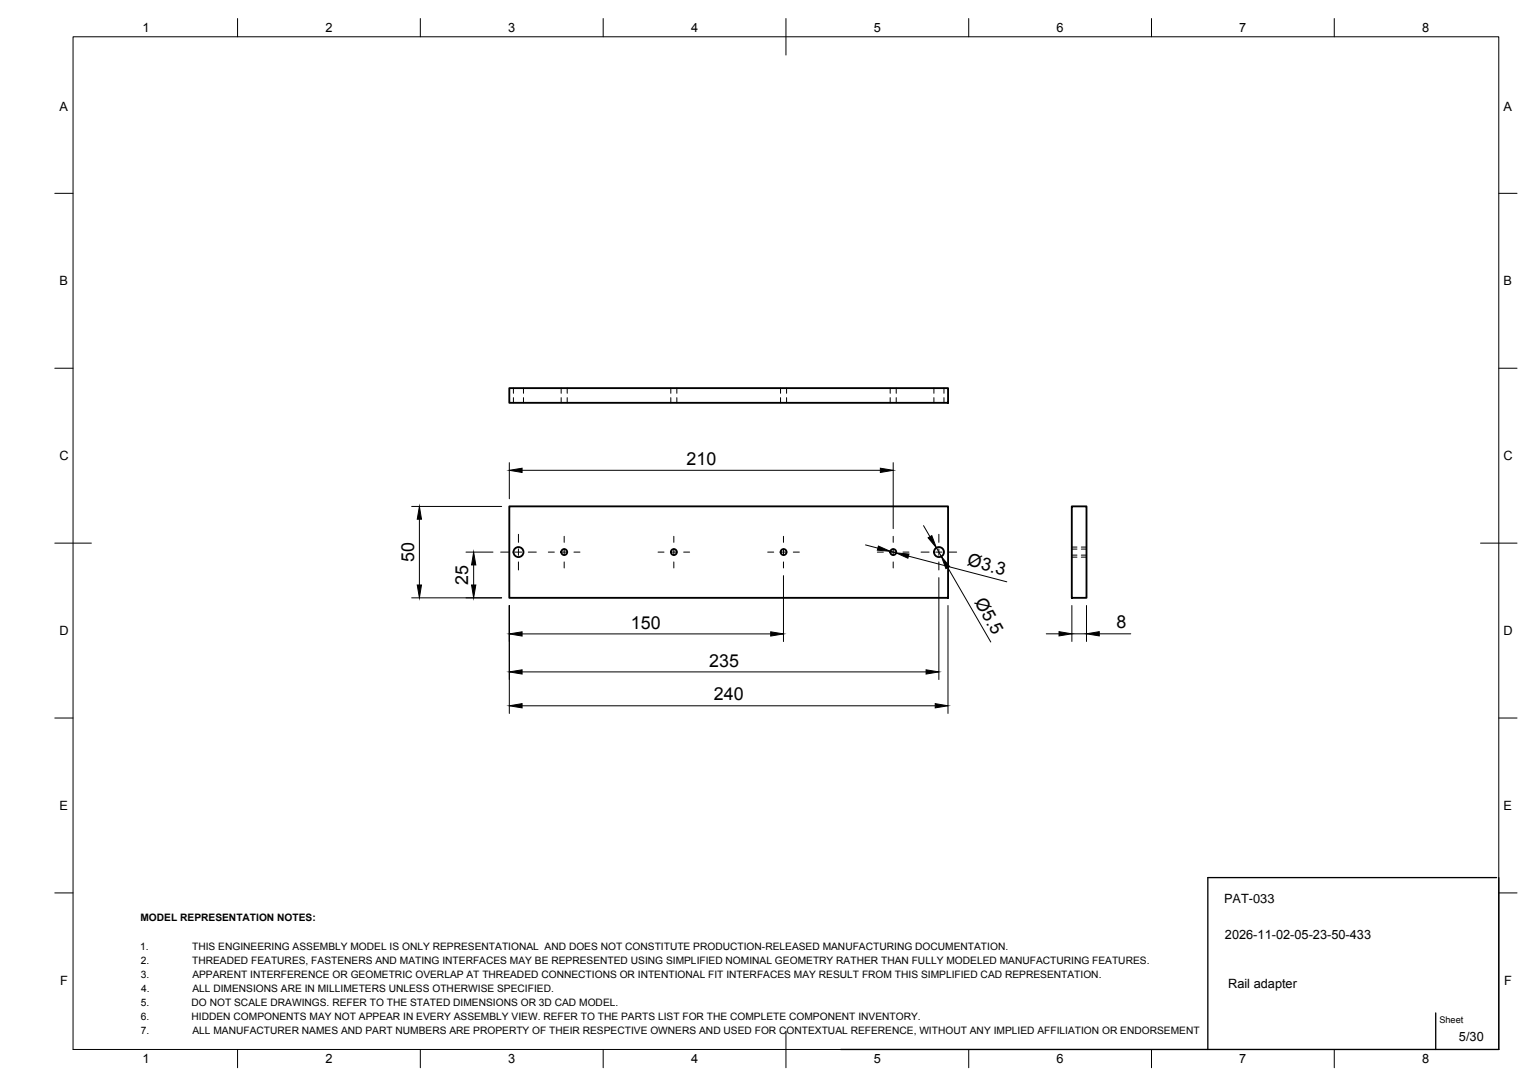
ISO-10303-21;
HEADER;
/* Generated by software containing ST-Developer
 * from STEP Tools, Inc. (www.steptools.com) 
 */

FILE_DESCRIPTION(
/* description */ ('Dual-rail gantry carriage'),
/* implementation_level */ '2;1');

FILE_NAME(
/* name */ 'Rail adapter.step',
/* time_stamp */ '2026-10-27T10:49:15-07:00',
/* author */ (''),
/* organization */ (''),
/* preprocessor_version */ 'ST-DEVELOPER v20.2',
/* originating_system */ 'Autodesk Translation Framework v15.17.0.0',
/* authorisation */ '');

FILE_SCHEMA (('AUTOMOTIVE_DESIGN { 1 0 10303 214 3 1 1 }'));
ENDSEC;

DATA;
#10=MECHANICAL_DESIGN_GEOMETRIC_PRESENTATION_REPRESENTATION('',(#585),#12804);
#523=SHAPE_REPRESENTATION_RELATIONSHIP('SRR','None',#13001,#554);
#554=ADVANCED_BREP_SHAPE_REPRESENTATION('',(#616),#12771);
#585=STYLED_ITEM('',(#13240),#616);
#616=MANIFOLD_SOLID_BREP('Body1',#7363);
#642=FACE_BOUND('',#1448,.T.);
#643=FACE_BOUND('',#1449,.T.);
#644=FACE_BOUND('',#1450,.T.);
#645=FACE_BOUND('',#1451,.T.);
#646=FACE_BOUND('',#1452,.T.);
#647=FACE_BOUND('',#1453,.T.);
#648=FACE_BOUND('',#1455,.T.);
#649=FACE_BOUND('',#1456,.T.);
#650=FACE_BOUND('',#1457,.T.);
#651=FACE_BOUND('',#1458,.T.);
#652=FACE_BOUND('',#1459,.T.);
#653=FACE_BOUND('',#1460,.T.);
#764=PLANE('',#7762);
#765=PLANE('',#7763);
#766=PLANE('',#7764);
#767=PLANE('',#7765);
#768=PLANE('',#7766);
#769=PLANE('',#7767);
#1048=FACE_OUTER_BOUND('',#1437,.T.);
#1049=FACE_OUTER_BOUND('',#1438,.T.);
#1050=FACE_OUTER_BOUND('',#1439,.T.);
#1051=FACE_OUTER_BOUND('',#1440,.T.);
#1052=FACE_OUTER_BOUND('',#1441,.T.);
#1053=FACE_OUTER_BOUND('',#1442,.T.);
#1054=FACE_OUTER_BOUND('',#1443,.T.);
#1055=FACE_OUTER_BOUND('',#1444,.T.);
#1056=FACE_OUTER_BOUND('',#1445,.T.);
#1057=FACE_OUTER_BOUND('',#1446,.T.);
#1058=FACE_OUTER_BOUND('',#1447,.T.);
#1059=FACE_OUTER_BOUND('',#1454,.T.);
#1437=EDGE_LOOP('',(#5067,#5068,#5069,#5070));
#1438=EDGE_LOOP('',(#5071,#5072,#5073,#5074));
#1439=EDGE_LOOP('',(#5075,#5076,#5077,#5078));
#1440=EDGE_LOOP('',(#5079,#5080,#5081,#5082));
#1441=EDGE_LOOP('',(#5083,#5084,#5085,#5086));
#1442=EDGE_LOOP('',(#5087,#5088,#5089,#5090));
#1443=EDGE_LOOP('',(#5091,#5092,#5093,#5094));
#1444=EDGE_LOOP('',(#5095,#5096,#5097,#5098));
#1445=EDGE_LOOP('',(#5099,#5100,#5101,#5102));
#1446=EDGE_LOOP('',(#5103,#5104,#5105,#5106));
#1447=EDGE_LOOP('',(#5107,#5108,#5109,#5110));
#1448=EDGE_LOOP('',(#5111));
#1449=EDGE_LOOP('',(#5112));
#1450=EDGE_LOOP('',(#5113));
#1451=EDGE_LOOP('',(#5114));
#1452=EDGE_LOOP('',(#5115));
#1453=EDGE_LOOP('',(#5116));
#1454=EDGE_LOOP('',(#5117,#5118,#5119,#5120));
#1455=EDGE_LOOP('',(#5121));
#1456=EDGE_LOOP('',(#5122));
#1457=EDGE_LOOP('',(#5123));
#1458=EDGE_LOOP('',(#5124));
#1459=EDGE_LOOP('',(#5125));
#1460=EDGE_LOOP('',(#5126));
#1948=LINE('',#10695,#2657);
#1949=LINE('',#10701,#2658);
#1950=LINE('',#10707,#2659);
#1951=LINE('',#10713,#2660);
#1952=LINE('',#10719,#2661);
#1953=LINE('',#10725,#2662);
#1954=LINE('',#10730,#2663);
#1955=LINE('',#10732,#2664);
#1956=LINE('',#10734,#2665);
#1957=LINE('',#10735,#2666);
#1958=LINE('',#10738,#2667);
#1959=LINE('',#10740,#2668);
#1960=LINE('',#10741,#2669);
#1961=LINE('',#10744,#2670);
#1962=LINE('',#10746,#2671);
#1963=LINE('',#10747,#2672);
#1964=LINE('',#10749,#2673);
#1965=LINE('',#10750,#2674);
#2657=VECTOR('',#8497,0.164999999999999);
#2658=VECTOR('',#8504,0.164999999999999);
#2659=VECTOR('',#8511,0.164999999999999);
#2660=VECTOR('',#8518,0.164999999999999);
#2661=VECTOR('',#8525,0.275);
#2662=VECTOR('',#8532,0.274999999999999);
#2663=VECTOR('',#8537,1.);
#2664=VECTOR('',#8538,1.);
#2665=VECTOR('',#8539,1.);
#2666=VECTOR('',#8540,1.);
#2667=VECTOR('',#8543,1.);
#2668=VECTOR('',#8544,1.);
#2669=VECTOR('',#8545,1.);
#2670=VECTOR('',#8548,1.);
#2671=VECTOR('',#8549,1.);
#2672=VECTOR('',#8550,1.);
#2673=VECTOR('',#8553,1.);
#2674=VECTOR('',#8554,1.);
#3366=CIRCLE('',#7745,0.164999999999999);
#3367=CIRCLE('',#7746,0.164999999999999);
#3368=CIRCLE('',#7748,0.164999999999999);
#3369=CIRCLE('',#7749,0.164999999999999);
#3370=CIRCLE('',#7751,0.164999999999999);
#3371=CIRCLE('',#7752,0.164999999999999);
#3372=CIRCLE('',#7754,0.164999999999999);
#3373=CIRCLE('',#7755,0.164999999999999);
#3374=CIRCLE('',#7757,0.275);
#3375=CIRCLE('',#7758,0.275);
#3376=CIRCLE('',#7760,0.274999999999999);
#3377=CIRCLE('',#7761,0.274999999999999);
#3566=VERTEX_POINT('',#10692);
#3567=VERTEX_POINT('',#10694);
#3568=VERTEX_POINT('',#10698);
#3569=VERTEX_POINT('',#10700);
#3570=VERTEX_POINT('',#10704);
#3571=VERTEX_POINT('',#10706);
#3572=VERTEX_POINT('',#10710);
#3573=VERTEX_POINT('',#10712);
#3574=VERTEX_POINT('',#10716);
#3575=VERTEX_POINT('',#10718);
#3576=VERTEX_POINT('',#10722);
#3577=VERTEX_POINT('',#10724);
#3578=VERTEX_POINT('',#10728);
#3579=VERTEX_POINT('',#10729);
#3580=VERTEX_POINT('',#10731);
#3581=VERTEX_POINT('',#10733);
#3582=VERTEX_POINT('',#10737);
#3583=VERTEX_POINT('',#10739);
#3584=VERTEX_POINT('',#10743);
#3585=VERTEX_POINT('',#10745);
#4156=EDGE_CURVE('',#3566,#3566,#3366,.T.);
#4157=EDGE_CURVE('',#3566,#3567,#1948,.T.);
#4158=EDGE_CURVE('',#3567,#3567,#3367,.T.);
#4159=EDGE_CURVE('',#3568,#3568,#3368,.T.);
#4160=EDGE_CURVE('',#3568,#3569,#1949,.T.);
#4161=EDGE_CURVE('',#3569,#3569,#3369,.T.);
#4162=EDGE_CURVE('',#3570,#3570,#3370,.T.);
#4163=EDGE_CURVE('',#3570,#3571,#1950,.T.);
#4164=EDGE_CURVE('',#3571,#3571,#3371,.T.);
#4165=EDGE_CURVE('',#3572,#3572,#3372,.T.);
#4166=EDGE_CURVE('',#3572,#3573,#1951,.T.);
#4167=EDGE_CURVE('',#3573,#3573,#3373,.T.);
#4168=EDGE_CURVE('',#3574,#3574,#3374,.T.);
#4169=EDGE_CURVE('',#3574,#3575,#1952,.T.);
#4170=EDGE_CURVE('',#3575,#3575,#3375,.T.);
#4171=EDGE_CURVE('',#3576,#3576,#3376,.T.);
#4172=EDGE_CURVE('',#3576,#3577,#1953,.T.);
#4173=EDGE_CURVE('',#3577,#3577,#3377,.T.);
#4174=EDGE_CURVE('',#3578,#3579,#1954,.T.);
#4175=EDGE_CURVE('',#3579,#3580,#1955,.T.);
#4176=EDGE_CURVE('',#3581,#3580,#1956,.T.);
#4177=EDGE_CURVE('',#3578,#3581,#1957,.T.);
#4178=EDGE_CURVE('',#3582,#3578,#1958,.T.);
#4179=EDGE_CURVE('',#3583,#3581,#1959,.T.);
#4180=EDGE_CURVE('',#3582,#3583,#1960,.T.);
#4181=EDGE_CURVE('',#3584,#3582,#1961,.T.);
#4182=EDGE_CURVE('',#3585,#3583,#1962,.T.);
#4183=EDGE_CURVE('',#3584,#3585,#1963,.T.);
#4184=EDGE_CURVE('',#3579,#3584,#1964,.T.);
#4185=EDGE_CURVE('',#3580,#3585,#1965,.T.);
#5067=ORIENTED_EDGE('',*,*,#4156,.F.);
#5068=ORIENTED_EDGE('',*,*,#4157,.T.);
#5069=ORIENTED_EDGE('',*,*,#4158,.F.);
#5070=ORIENTED_EDGE('',*,*,#4157,.F.);
#5071=ORIENTED_EDGE('',*,*,#4159,.F.);
#5072=ORIENTED_EDGE('',*,*,#4160,.T.);
#5073=ORIENTED_EDGE('',*,*,#4161,.F.);
#5074=ORIENTED_EDGE('',*,*,#4160,.F.);
#5075=ORIENTED_EDGE('',*,*,#4162,.F.);
#5076=ORIENTED_EDGE('',*,*,#4163,.T.);
#5077=ORIENTED_EDGE('',*,*,#4164,.F.);
#5078=ORIENTED_EDGE('',*,*,#4163,.F.);
#5079=ORIENTED_EDGE('',*,*,#4165,.F.);
#5080=ORIENTED_EDGE('',*,*,#4166,.T.);
#5081=ORIENTED_EDGE('',*,*,#4167,.F.);
#5082=ORIENTED_EDGE('',*,*,#4166,.F.);
#5083=ORIENTED_EDGE('',*,*,#4168,.F.);
#5084=ORIENTED_EDGE('',*,*,#4169,.T.);
#5085=ORIENTED_EDGE('',*,*,#4170,.F.);
#5086=ORIENTED_EDGE('',*,*,#4169,.F.);
#5087=ORIENTED_EDGE('',*,*,#4171,.F.);
#5088=ORIENTED_EDGE('',*,*,#4172,.T.);
#5089=ORIENTED_EDGE('',*,*,#4173,.F.);
#5090=ORIENTED_EDGE('',*,*,#4172,.F.);
#5091=ORIENTED_EDGE('',*,*,#4174,.T.);
#5092=ORIENTED_EDGE('',*,*,#4175,.T.);
#5093=ORIENTED_EDGE('',*,*,#4176,.F.);
#5094=ORIENTED_EDGE('',*,*,#4177,.F.);
#5095=ORIENTED_EDGE('',*,*,#4178,.T.);
#5096=ORIENTED_EDGE('',*,*,#4177,.T.);
#5097=ORIENTED_EDGE('',*,*,#4179,.F.);
#5098=ORIENTED_EDGE('',*,*,#4180,.F.);
#5099=ORIENTED_EDGE('',*,*,#4181,.T.);
#5100=ORIENTED_EDGE('',*,*,#4180,.T.);
#5101=ORIENTED_EDGE('',*,*,#4182,.F.);
#5102=ORIENTED_EDGE('',*,*,#4183,.F.);
#5103=ORIENTED_EDGE('',*,*,#4184,.T.);
#5104=ORIENTED_EDGE('',*,*,#4183,.T.);
#5105=ORIENTED_EDGE('',*,*,#4185,.F.);
#5106=ORIENTED_EDGE('',*,*,#4175,.F.);
#5107=ORIENTED_EDGE('',*,*,#4185,.T.);
#5108=ORIENTED_EDGE('',*,*,#4182,.T.);
#5109=ORIENTED_EDGE('',*,*,#4179,.T.);
#5110=ORIENTED_EDGE('',*,*,#4176,.T.);
#5111=ORIENTED_EDGE('',*,*,#4173,.T.);
#5112=ORIENTED_EDGE('',*,*,#4170,.T.);
#5113=ORIENTED_EDGE('',*,*,#4167,.T.);
#5114=ORIENTED_EDGE('',*,*,#4164,.T.);
#5115=ORIENTED_EDGE('',*,*,#4161,.T.);
#5116=ORIENTED_EDGE('',*,*,#4158,.T.);
#5117=ORIENTED_EDGE('',*,*,#4184,.F.);
#5118=ORIENTED_EDGE('',*,*,#4174,.F.);
#5119=ORIENTED_EDGE('',*,*,#4178,.F.);
#5120=ORIENTED_EDGE('',*,*,#4181,.F.);
#5121=ORIENTED_EDGE('',*,*,#4171,.T.);
#5122=ORIENTED_EDGE('',*,*,#4168,.T.);
#5123=ORIENTED_EDGE('',*,*,#4165,.T.);
#5124=ORIENTED_EDGE('',*,*,#4162,.T.);
#5125=ORIENTED_EDGE('',*,*,#4159,.T.);
#5126=ORIENTED_EDGE('',*,*,#4156,.T.);
#6889=CYLINDRICAL_SURFACE('',#7744,0.164999999999999);
#6890=CYLINDRICAL_SURFACE('',#7747,0.164999999999999);
#6891=CYLINDRICAL_SURFACE('',#7750,0.164999999999999);
#6892=CYLINDRICAL_SURFACE('',#7753,0.164999999999999);
#6893=CYLINDRICAL_SURFACE('',#7756,0.275);
#6894=CYLINDRICAL_SURFACE('',#7759,0.274999999999999);
#6974=ADVANCED_FACE('',(#1048),#6889,.F.);
#6975=ADVANCED_FACE('',(#1049),#6890,.F.);
#6976=ADVANCED_FACE('',(#1050),#6891,.F.);
#6977=ADVANCED_FACE('',(#1051),#6892,.F.);
#6978=ADVANCED_FACE('',(#1052),#6893,.F.);
#6979=ADVANCED_FACE('',(#1053),#6894,.F.);
#6980=ADVANCED_FACE('',(#1054),#764,.T.);
#6981=ADVANCED_FACE('',(#1055),#765,.T.);
#6982=ADVANCED_FACE('',(#1056),#766,.T.);
#6983=ADVANCED_FACE('',(#1057),#767,.T.);
#6984=ADVANCED_FACE('',(#1058,#642,#643,#644,#645,#646,#647),#768,.T.);
#6985=ADVANCED_FACE('',(#1059,#648,#649,#650,#651,#652,#653),#769,.F.);
#7363=CLOSED_SHELL('',(#6974,#6975,#6976,#6977,#6978,#6979,#6980,#6981,
#6982,#6983,#6984,#6985));
#7743=AXIS2_PLACEMENT_3D('',#10690,#8491,#8492);
#7744=AXIS2_PLACEMENT_3D('',#10691,#8493,#8494);
#7745=AXIS2_PLACEMENT_3D('',#10693,#8495,#8496);
#7746=AXIS2_PLACEMENT_3D('',#10696,#8498,#8499);
#7747=AXIS2_PLACEMENT_3D('',#10697,#8500,#8501);
#7748=AXIS2_PLACEMENT_3D('',#10699,#8502,#8503);
#7749=AXIS2_PLACEMENT_3D('',#10702,#8505,#8506);
#7750=AXIS2_PLACEMENT_3D('',#10703,#8507,#8508);
#7751=AXIS2_PLACEMENT_3D('',#10705,#8509,#8510);
#7752=AXIS2_PLACEMENT_3D('',#10708,#8512,#8513);
#7753=AXIS2_PLACEMENT_3D('',#10709,#8514,#8515);
#7754=AXIS2_PLACEMENT_3D('',#10711,#8516,#8517);
#7755=AXIS2_PLACEMENT_3D('',#10714,#8519,#8520);
#7756=AXIS2_PLACEMENT_3D('',#10715,#8521,#8522);
#7757=AXIS2_PLACEMENT_3D('',#10717,#8523,#8524);
#7758=AXIS2_PLACEMENT_3D('',#10720,#8526,#8527);
#7759=AXIS2_PLACEMENT_3D('',#10721,#8528,#8529);
#7760=AXIS2_PLACEMENT_3D('',#10723,#8530,#8531);
#7761=AXIS2_PLACEMENT_3D('',#10726,#8533,#8534);
#7762=AXIS2_PLACEMENT_3D('',#10727,#8535,#8536);
#7763=AXIS2_PLACEMENT_3D('',#10736,#8541,#8542);
#7764=AXIS2_PLACEMENT_3D('',#10742,#8546,#8547);
#7765=AXIS2_PLACEMENT_3D('',#10748,#8551,#8552);
#7766=AXIS2_PLACEMENT_3D('',#10751,#8555,#8556);
#7767=AXIS2_PLACEMENT_3D('',#10752,#8557,#8558);
#8491=DIRECTION('axis',(0.,0.,1.));
#8492=DIRECTION('refdir',(1.,0.,0.));
#8493=DIRECTION('center_axis',(0.,0.,1.));
#8494=DIRECTION('ref_axis',(1.,0.,0.));
#8495=DIRECTION('center_axis',(0.,0.,1.));
#8496=DIRECTION('ref_axis',(1.,0.,0.));
#8497=DIRECTION('',(0.,0.,1.));
#8498=DIRECTION('center_axis',(0.,0.,-1.));
#8499=DIRECTION('ref_axis',(1.,0.,0.));
#8500=DIRECTION('center_axis',(0.,0.,1.));
#8501=DIRECTION('ref_axis',(1.,0.,0.));
#8502=DIRECTION('center_axis',(0.,0.,1.));
#8503=DIRECTION('ref_axis',(1.,0.,0.));
#8504=DIRECTION('',(0.,0.,1.));
#8505=DIRECTION('center_axis',(0.,0.,-1.));
#8506=DIRECTION('ref_axis',(1.,0.,0.));
#8507=DIRECTION('center_axis',(0.,0.,1.));
#8508=DIRECTION('ref_axis',(1.,0.,0.));
#8509=DIRECTION('center_axis',(0.,0.,1.));
#8510=DIRECTION('ref_axis',(1.,0.,0.));
#8511=DIRECTION('',(0.,0.,1.));
#8512=DIRECTION('center_axis',(0.,0.,-1.));
#8513=DIRECTION('ref_axis',(1.,0.,0.));
#8514=DIRECTION('center_axis',(0.,0.,1.));
#8515=DIRECTION('ref_axis',(1.,0.,0.));
#8516=DIRECTION('center_axis',(0.,0.,1.));
#8517=DIRECTION('ref_axis',(1.,0.,0.));
#8518=DIRECTION('',(0.,0.,1.));
#8519=DIRECTION('center_axis',(0.,0.,-1.));
#8520=DIRECTION('ref_axis',(1.,0.,0.));
#8521=DIRECTION('center_axis',(0.,0.,1.));
#8522=DIRECTION('ref_axis',(1.,0.,0.));
#8523=DIRECTION('center_axis',(0.,0.,1.));
#8524=DIRECTION('ref_axis',(1.,0.,0.));
#8525=DIRECTION('',(0.,0.,1.));
#8526=DIRECTION('center_axis',(0.,0.,-1.));
#8527=DIRECTION('ref_axis',(1.,0.,0.));
#8528=DIRECTION('center_axis',(0.,0.,1.));
#8529=DIRECTION('ref_axis',(1.,0.,0.));
#8530=DIRECTION('center_axis',(0.,0.,1.));
#8531=DIRECTION('ref_axis',(1.,0.,0.));
#8532=DIRECTION('',(0.,0.,1.));
#8533=DIRECTION('center_axis',(0.,0.,-1.));
#8534=DIRECTION('ref_axis',(1.,0.,0.));
#8535=DIRECTION('center_axis',(0.,1.,0.));
#8536=DIRECTION('ref_axis',(-1.,0.,0.));
#8537=DIRECTION('',(-1.,0.,0.));
#8538=DIRECTION('',(0.,0.,1.));
#8539=DIRECTION('',(-1.,0.,0.));
#8540=DIRECTION('',(0.,0.,1.));
#8541=DIRECTION('center_axis',(1.,0.,0.));
#8542=DIRECTION('ref_axis',(0.,1.,0.));
#8543=DIRECTION('',(0.,1.,0.));
#8544=DIRECTION('',(0.,1.,0.));
#8545=DIRECTION('',(0.,0.,1.));
#8546=DIRECTION('center_axis',(0.,-1.,0.));
#8547=DIRECTION('ref_axis',(1.,0.,0.));
#8548=DIRECTION('',(1.,0.,0.));
#8549=DIRECTION('',(1.,0.,0.));
#8550=DIRECTION('',(0.,0.,1.));
#8551=DIRECTION('center_axis',(-1.,0.,0.));
#8552=DIRECTION('ref_axis',(0.,-1.,0.));
#8553=DIRECTION('',(0.,-1.,0.));
#8554=DIRECTION('',(0.,-1.,0.));
#8555=DIRECTION('center_axis',(0.,0.,1.));
#8556=DIRECTION('ref_axis',(1.,0.,0.));
#8557=DIRECTION('center_axis',(0.,0.,1.));
#8558=DIRECTION('ref_axis',(1.,0.,0.));
#10690=CARTESIAN_POINT('',(0.,0.,0.));
#10691=CARTESIAN_POINT('Origin',(23.,-10.,1.9));
#10692=CARTESIAN_POINT('',(22.835,-10.,2.));
#10693=CARTESIAN_POINT('Origin',(23.,-10.,2.));
#10694=CARTESIAN_POINT('',(22.835,-10.,2.8));
#10695=CARTESIAN_POINT('',(22.835,-10.,1.9));
#10696=CARTESIAN_POINT('Origin',(23.,-10.,2.8));
#10697=CARTESIAN_POINT('Origin',(17.,-10.,1.9));
#10698=CARTESIAN_POINT('',(16.835,-10.,2.));
#10699=CARTESIAN_POINT('Origin',(17.,-10.,2.));
#10700=CARTESIAN_POINT('',(16.835,-10.,2.8));
#10701=CARTESIAN_POINT('',(16.835,-10.,1.9));
#10702=CARTESIAN_POINT('Origin',(17.,-10.,2.8));
#10703=CARTESIAN_POINT('Origin',(11.,-10.,1.9));
#10704=CARTESIAN_POINT('',(10.835,-10.,2.));
#10705=CARTESIAN_POINT('Origin',(11.,-10.,2.));
#10706=CARTESIAN_POINT('',(10.835,-10.,2.8));
#10707=CARTESIAN_POINT('',(10.835,-10.,1.9));
#10708=CARTESIAN_POINT('Origin',(11.,-10.,2.8));
#10709=CARTESIAN_POINT('Origin',(29.,-10.,1.9));
#10710=CARTESIAN_POINT('',(28.835,-10.,2.));
#10711=CARTESIAN_POINT('Origin',(29.,-10.,2.));
#10712=CARTESIAN_POINT('',(28.835,-10.,2.8));
#10713=CARTESIAN_POINT('',(28.835,-10.,1.9));
#10714=CARTESIAN_POINT('Origin',(29.,-10.,2.8));
#10715=CARTESIAN_POINT('Origin',(8.5,-10.,1.9));
#10716=CARTESIAN_POINT('',(8.225,-10.,2.));
#10717=CARTESIAN_POINT('Origin',(8.5,-10.,2.));
#10718=CARTESIAN_POINT('',(8.225,-10.,2.8));
#10719=CARTESIAN_POINT('',(8.225,-10.,1.9));
#10720=CARTESIAN_POINT('Origin',(8.5,-10.,2.8));
#10721=CARTESIAN_POINT('Origin',(31.5,-10.,1.9));
#10722=CARTESIAN_POINT('',(31.225,-10.,2.));
#10723=CARTESIAN_POINT('Origin',(31.5,-10.,2.));
#10724=CARTESIAN_POINT('',(31.225,-10.,2.8));
#10725=CARTESIAN_POINT('',(31.225,-10.,1.9));
#10726=CARTESIAN_POINT('Origin',(31.5,-10.,2.8));
#10727=CARTESIAN_POINT('Origin',(32.,-7.5,2.));
#10728=CARTESIAN_POINT('',(32.,-7.5,2.));
#10729=CARTESIAN_POINT('',(8.,-7.5,2.));
#10730=CARTESIAN_POINT('',(32.,-7.5,2.));
#10731=CARTESIAN_POINT('',(8.,-7.5,2.8));
#10732=CARTESIAN_POINT('',(8.,-7.5,2.));
#10733=CARTESIAN_POINT('',(32.,-7.5,2.8));
#10734=CARTESIAN_POINT('',(32.,-7.5,2.8));
#10735=CARTESIAN_POINT('',(32.,-7.5,2.));
#10736=CARTESIAN_POINT('Origin',(32.,-12.5,2.));
#10737=CARTESIAN_POINT('',(32.,-12.5,2.));
#10738=CARTESIAN_POINT('',(32.,-12.5,2.));
#10739=CARTESIAN_POINT('',(32.,-12.5,2.8));
#10740=CARTESIAN_POINT('',(32.,-12.5,2.8));
#10741=CARTESIAN_POINT('',(32.,-12.5,2.));
#10742=CARTESIAN_POINT('Origin',(8.,-12.5,2.));
#10743=CARTESIAN_POINT('',(8.,-12.5,2.));
#10744=CARTESIAN_POINT('',(8.,-12.5,2.));
#10745=CARTESIAN_POINT('',(8.,-12.5,2.8));
#10746=CARTESIAN_POINT('',(8.,-12.5,2.8));
#10747=CARTESIAN_POINT('',(8.,-12.5,2.));
#10748=CARTESIAN_POINT('Origin',(8.,-7.5,2.));
#10749=CARTESIAN_POINT('',(8.,-7.5,2.));
#10750=CARTESIAN_POINT('',(8.,-7.5,2.8));
#10751=CARTESIAN_POINT('Origin',(20.,-10.,2.8));
#10752=CARTESIAN_POINT('Origin',(20.,-10.,2.));
#12735=UNCERTAINTY_MEASURE_WITH_UNIT(LENGTH_MEASURE(0.001),#12805,
'DISTANCE_ACCURACY_VALUE',
'Maximum model space distance between geometric entities at asserted c
onnectivities');
#12768=UNCERTAINTY_MEASURE_WITH_UNIT(LENGTH_MEASURE(0.001),#12805,
'DISTANCE_ACCURACY_VALUE',
'Maximum model space distance between geometric entities at asserted c
onnectivities');
#12771=(
GEOMETRIC_REPRESENTATION_CONTEXT(3)
GLOBAL_UNCERTAINTY_ASSIGNED_CONTEXT((#12735))
GLOBAL_UNIT_ASSIGNED_CONTEXT((#12805,#12807,#12808))
REPRESENTATION_CONTEXT('','3D')
);
#12804=(
GEOMETRIC_REPRESENTATION_CONTEXT(3)
GLOBAL_UNCERTAINTY_ASSIGNED_CONTEXT((#12768))
GLOBAL_UNIT_ASSIGNED_CONTEXT((#12805,#12807,#12808))
REPRESENTATION_CONTEXT('','3D')
);
#12805=(
LENGTH_UNIT()
NAMED_UNIT(*)
SI_UNIT(.CENTI.,.METRE.)
);
#12807=(
NAMED_UNIT(*)
PLANE_ANGLE_UNIT()
SI_UNIT($,.RADIAN.)
);
#12808=(
NAMED_UNIT(*)
SI_UNIT($,.STERADIAN.)
SOLID_ANGLE_UNIT()
);
#12811=SHAPE_DEFINITION_REPRESENTATION(#12846,#13001);
#12846=PRODUCT_DEFINITION_SHAPE('',$,#13037);
#13001=SHAPE_REPRESENTATION('',(#7743),#12771);
#13034=PRODUCT_DEFINITION_CONTEXT('part definition',#13141,'design');
#13037=PRODUCT_DEFINITION('Rail adapter','Rail adapter',#13072,#13034);
#13072=PRODUCT_DEFINITION_FORMATION('',$,#13145);
#13141=APPLICATION_CONTEXT(
'Core Data for Automotive Mechanical Design Process');
#13142=PRODUCT_CONTEXT('part definition',#13141,'mechanical');
#13145=PRODUCT('Rail adapter','Rail adapter','Rail adapter',(#13142));
#13234=COLOUR_RGB('Sky Blue',0.24,0.69,0.87);
#13235=FILL_AREA_STYLE_COLOUR('',#13234);
#13236=FILL_AREA_STYLE('',(#13235));
#13237=SURFACE_STYLE_FILL_AREA(#13236);
#13238=SURFACE_SIDE_STYLE('',(#13237));
#13239=SURFACE_STYLE_USAGE(.BOTH.,#13238);
#13240=PRESENTATION_STYLE_ASSIGNMENT((#13239));
ENDSEC;
END-ISO-10303-21;
